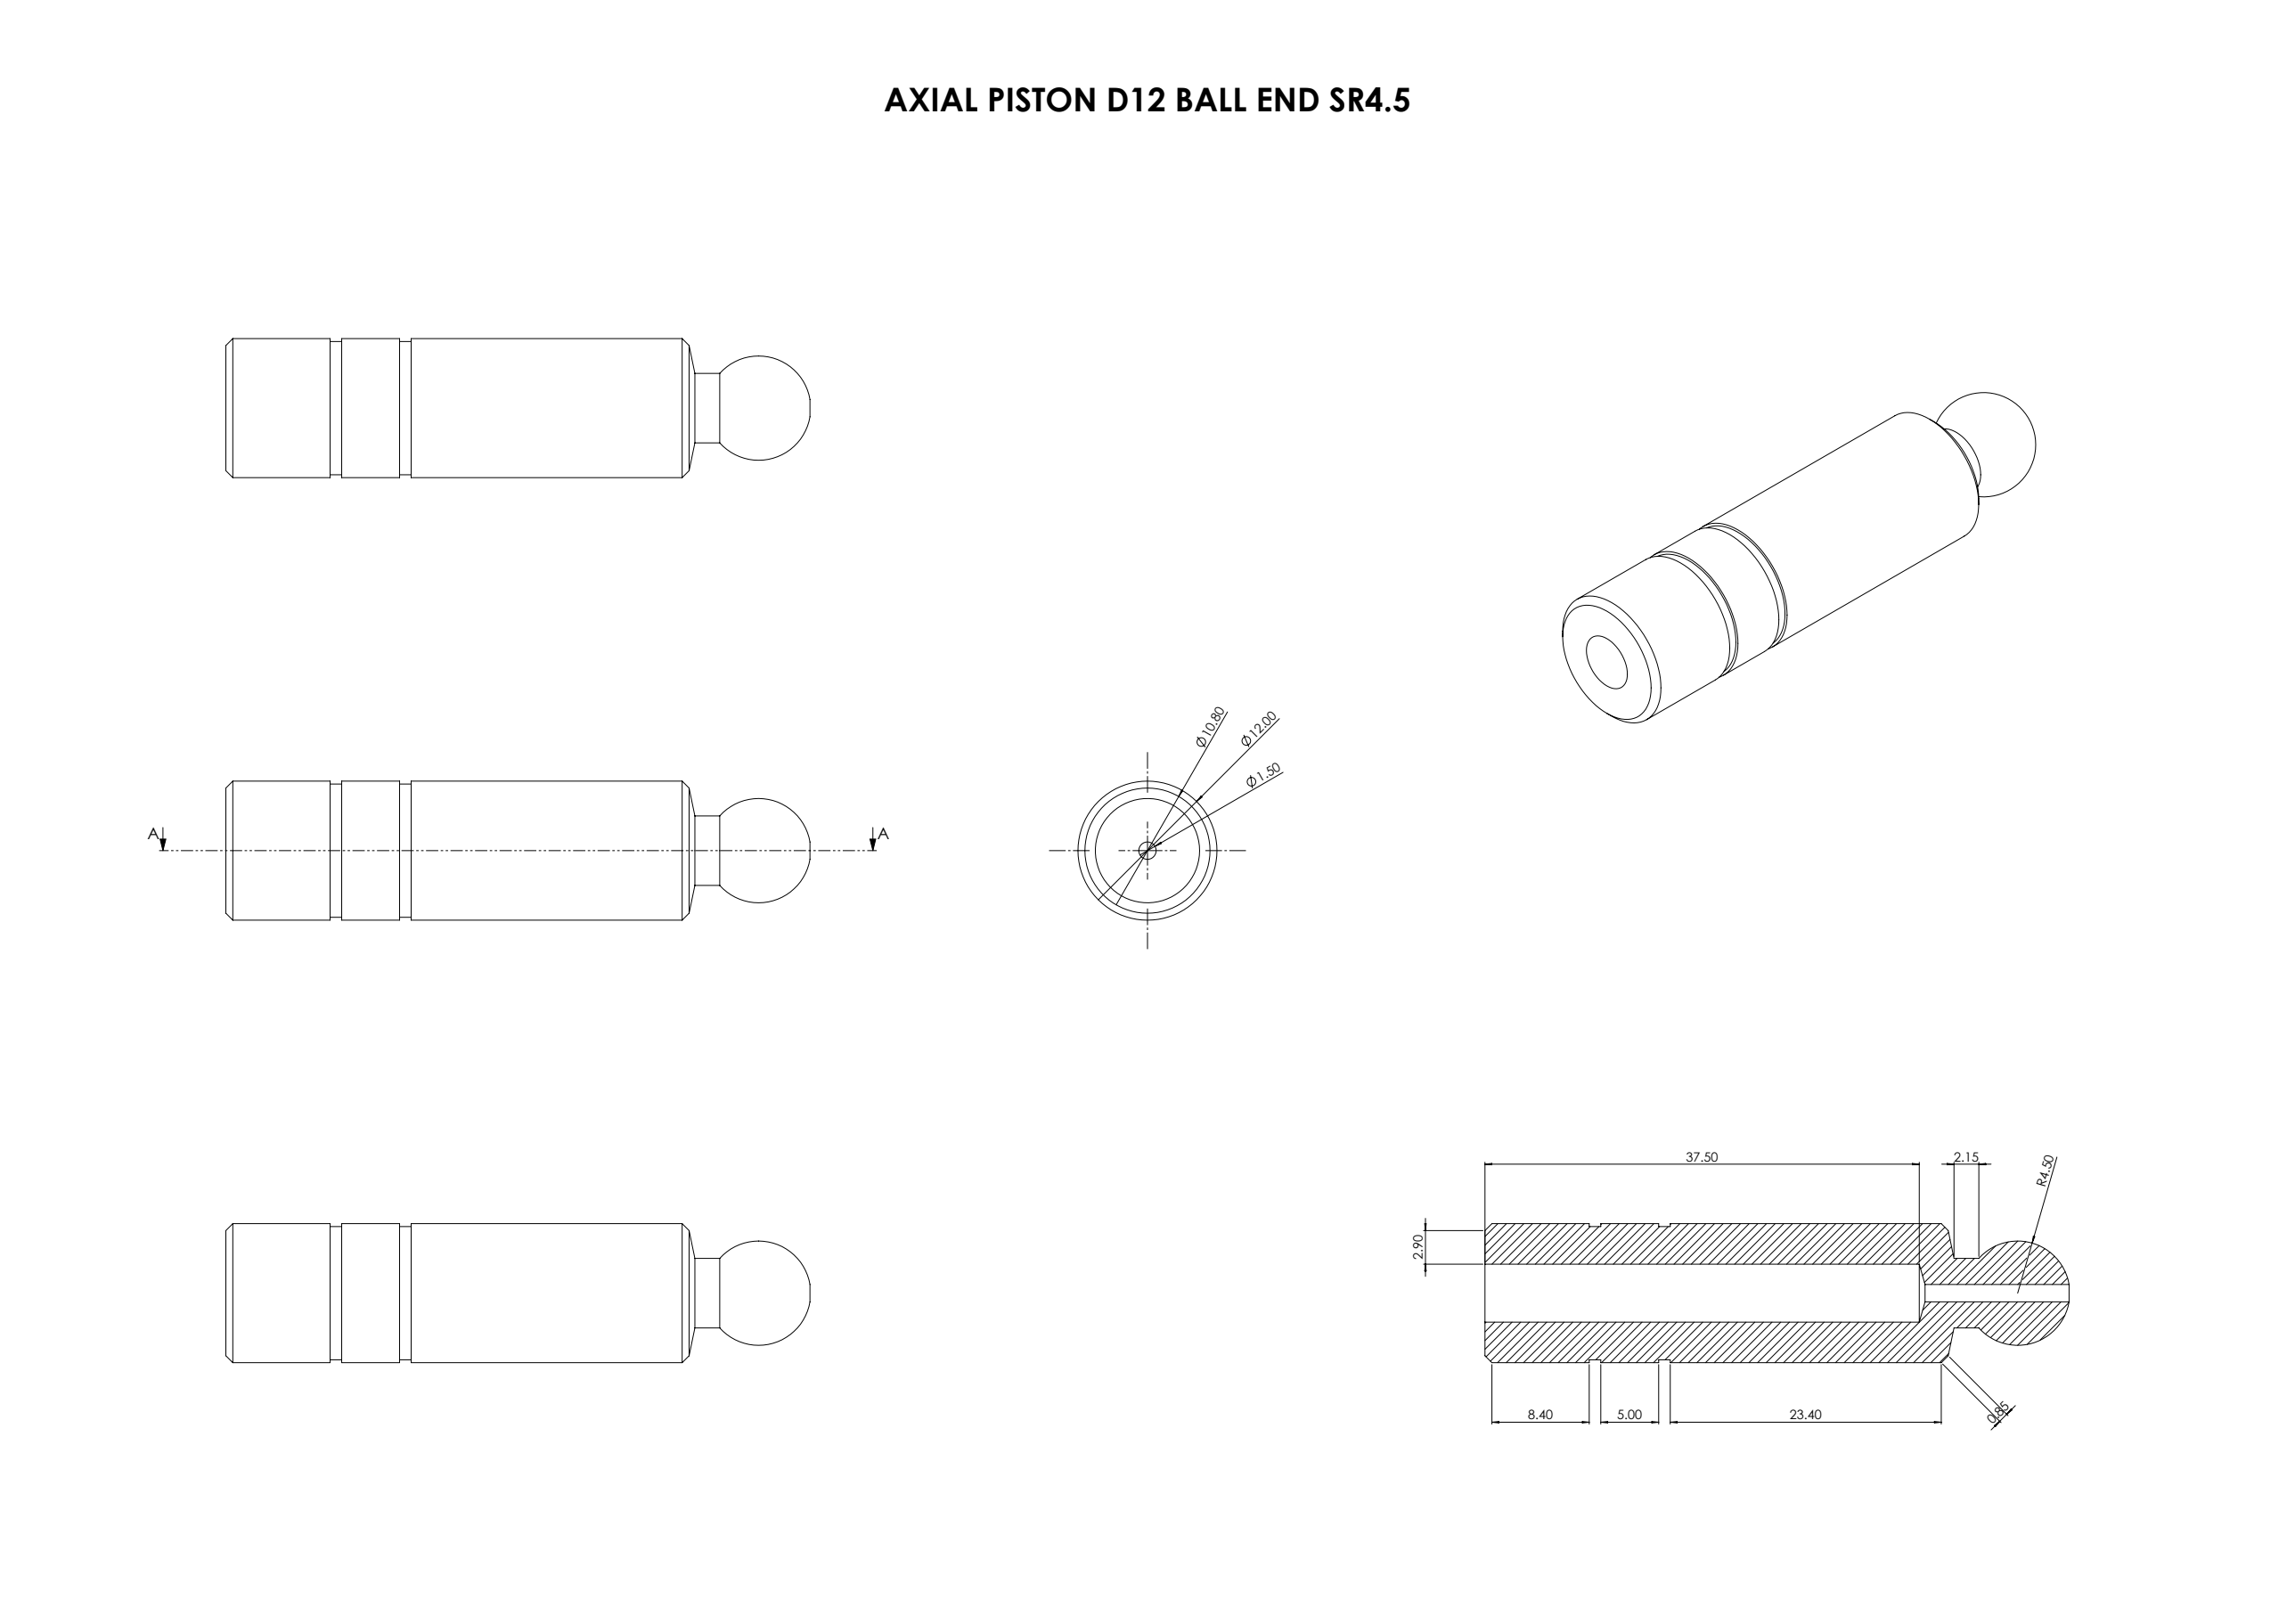
ISO-10303-21;
HEADER;
/* Generated by software containing ST-Developer
 * from STEP Tools, Inc. (www.steptools.com) 
 */

FILE_DESCRIPTION(
/* description */ (''),
/* implementation_level */ '2;1');

FILE_NAME(
/* name */ '06_Axial_Piston_D12_Ball_End_SR4.5.step',
/* time_stamp */ '2026-10-23T00:52:27+05:00',
/* author */ (''),
/* organization */ (''),
/* preprocessor_version */ 'ST-DEVELOPER v20.2',
/* originating_system */ 'Autodesk Translation Framework v15.15.0.0',
/* authorisation */ '');

FILE_SCHEMA (('AUTOMOTIVE_DESIGN { 1 0 10303 214 3 1 1 }'));
ENDSEC;

DATA;
#10=MECHANICAL_DESIGN_GEOMETRIC_PRESENTATION_REPRESENTATION('',(#1568),#59204);
#1521=SHAPE_REPRESENTATION_RELATIONSHIP('SRR','None',#59310,#1541);
#1541=ADVANCED_BREP_SHAPE_REPRESENTATION('',(#1588),#59197);
#1568=STYLED_ITEM('',(#59579),#1588);
#1588=MANIFOLD_SOLID_BREP('Piston',#22817);
#1597=SPHERICAL_SURFACE('',#24195,0.45);
#1747=FACE_BOUND('',#4969,.T.);
#1748=FACE_BOUND('',#4972,.T.);
#1749=FACE_BOUND('',#4975,.T.);
#1750=FACE_BOUND('',#4978,.T.);
#1751=FACE_BOUND('',#4986,.T.);
#2147=PLANE('',#24160);
#2148=PLANE('',#24165);
#2149=PLANE('',#24169);
#2150=PLANE('',#24173);
#2151=PLANE('',#24187);
#2565=CYLINDRICAL_SURFACE('',#24163,0.575);
#2566=CYLINDRICAL_SURFACE('',#24167,0.6);
#2567=CYLINDRICAL_SURFACE('',#24171,0.575);
#2568=CYLINDRICAL_SURFACE('',#24175,0.6);
#2569=CYLINDRICAL_SURFACE('',#24177,0.3);
#2570=CYLINDRICAL_SURFACE('',#24183,0.6);
#2571=CYLINDRICAL_SURFACE('',#24189,0.25);
#2572=CYLINDRICAL_SURFACE('',#24193,0.075);
#3515=FACE_OUTER_BOUND('',#4968,.T.);
#3516=FACE_OUTER_BOUND('',#4970,.T.);
#3517=FACE_OUTER_BOUND('',#4971,.T.);
#3518=FACE_OUTER_BOUND('',#4973,.T.);
#3519=FACE_OUTER_BOUND('',#4974,.T.);
#3520=FACE_OUTER_BOUND('',#4976,.T.);
#3521=FACE_OUTER_BOUND('',#4977,.T.);
#3522=FACE_OUTER_BOUND('',#4979,.T.);
#3523=FACE_OUTER_BOUND('',#4980,.T.);
#3524=FACE_OUTER_BOUND('',#4981,.T.);
#3525=FACE_OUTER_BOUND('',#4982,.T.);
#3526=FACE_OUTER_BOUND('',#4983,.T.);
#3527=FACE_OUTER_BOUND('',#4984,.T.);
#3528=FACE_OUTER_BOUND('',#4985,.T.);
#3529=FACE_OUTER_BOUND('',#4987,.T.);
#3530=FACE_OUTER_BOUND('',#4988,.T.);
#3531=FACE_OUTER_BOUND('',#4989,.T.);
#3532=FACE_OUTER_BOUND('',#4990,.T.);
#4968=EDGE_LOOP('',(#18954));
#4969=EDGE_LOOP('',(#18955));
#4970=EDGE_LOOP('',(#18956,#18957,#18958,#18959));
#4971=EDGE_LOOP('',(#18960));
#4972=EDGE_LOOP('',(#18961));
#4973=EDGE_LOOP('',(#18962,#18963,#18964,#18965));
#4974=EDGE_LOOP('',(#18966));
#4975=EDGE_LOOP('',(#18967));
#4976=EDGE_LOOP('',(#18968,#18969,#18970,#18971));
#4977=EDGE_LOOP('',(#18972));
#4978=EDGE_LOOP('',(#18973));
#4979=EDGE_LOOP('',(#18974,#18975,#18976,#18977));
#4980=EDGE_LOOP('',(#18978,#18979,#18980,#18981));
#4981=EDGE_LOOP('',(#18982,#18983,#18984,#18985));
#4982=EDGE_LOOP('',(#18986,#18987,#18988,#18989));
#4983=EDGE_LOOP('',(#18990,#18991,#18992,#18993));
#4984=EDGE_LOOP('',(#18994,#18995,#18996,#18997));
#4985=EDGE_LOOP('',(#18998));
#4986=EDGE_LOOP('',(#18999));
#4987=EDGE_LOOP('',(#19000,#19001,#19002,#19003));
#4988=EDGE_LOOP('',(#19004,#19005,#19006,#19007));
#4989=EDGE_LOOP('',(#19008,#19009,#19010,#19011));
#4990=EDGE_LOOP('',(#19012,#19013,#19014,#19015));
#6489=LINE('',#47284,#7922);
#6490=LINE('',#47290,#7923);
#6491=LINE('',#47298,#7924);
#6492=LINE('',#47304,#7925);
#6493=LINE('',#47310,#7926);
#6494=LINE('',#47315,#7927);
#6495=LINE('',#47317,#7928);
#6496=LINE('',#47321,#7929);
#6497=LINE('',#47325,#7930);
#6498=LINE('',#47331,#7931);
#6499=LINE('',#47335,#7932);
#6500=LINE('',#47339,#7933);
#7922=VECTOR('',#28355,0.575);
#7923=VECTOR('',#28362,0.6);
#7924=VECTOR('',#28373,0.575);
#7925=VECTOR('',#28380,0.6);
#7926=VECTOR('',#28387,0.3);
#7927=VECTOR('',#28394,0.42);
#7928=VECTOR('',#28397,0.57);
#7929=VECTOR('',#28402,0.6);
#7930=VECTOR('',#28407,0.57);
#7931=VECTOR('',#28414,0.25);
#7932=VECTOR('',#28419,0.1625);
#7933=VECTOR('',#28424,0.075);
#8855=CIRCLE('',#24161,0.6);
#8856=CIRCLE('',#24162,0.575);
#8857=CIRCLE('',#24164,0.575);
#8858=CIRCLE('',#24166,0.6);
#8859=CIRCLE('',#24168,0.6);
#8860=CIRCLE('',#24170,0.575);
#8861=CIRCLE('',#24172,0.575);
#8862=CIRCLE('',#24174,0.6);
#8863=CIRCLE('',#24176,0.6);
#8864=CIRCLE('',#24178,0.3);
#8865=CIRCLE('',#24179,0.3);
#8866=CIRCLE('',#24181,0.54);
#8867=CIRCLE('',#24184,0.6);
#8868=CIRCLE('',#24186,0.54);
#8869=CIRCLE('',#24188,0.25);
#8870=CIRCLE('',#24190,0.25);
#8871=CIRCLE('',#24192,0.075);
#8872=CIRCLE('',#24194,0.075);
#8873=CIRCLE('',#24196,0.45);
#10582=VERTEX_POINT('',#47277);
#10583=VERTEX_POINT('',#47279);
#10584=VERTEX_POINT('',#47282);
#10585=VERTEX_POINT('',#47286);
#10586=VERTEX_POINT('',#47289);
#10587=VERTEX_POINT('',#47293);
#10588=VERTEX_POINT('',#47296);
#10589=VERTEX_POINT('',#47300);
#10590=VERTEX_POINT('',#47303);
#10591=VERTEX_POINT('',#47307);
#10592=VERTEX_POINT('',#47309);
#10593=VERTEX_POINT('',#47313);
#10594=VERTEX_POINT('',#47319);
#10595=VERTEX_POINT('',#47323);
#10596=VERTEX_POINT('',#47327);
#10597=VERTEX_POINT('',#47330);
#10598=VERTEX_POINT('',#47334);
#10599=VERTEX_POINT('',#47338);
#13481=EDGE_CURVE('',#10582,#10582,#8855,.T.);
#13482=EDGE_CURVE('',#10583,#10583,#8856,.T.);
#13483=EDGE_CURVE('',#10584,#10584,#8857,.T.);
#13484=EDGE_CURVE('',#10584,#10583,#6489,.T.);
#13485=EDGE_CURVE('',#10585,#10585,#8858,.T.);
#13486=EDGE_CURVE('',#10585,#10586,#6490,.T.);
#13487=EDGE_CURVE('',#10586,#10586,#8859,.T.);
#13488=EDGE_CURVE('',#10587,#10587,#8860,.T.);
#13489=EDGE_CURVE('',#10588,#10588,#8861,.T.);
#13490=EDGE_CURVE('',#10588,#10587,#6491,.T.);
#13491=EDGE_CURVE('',#10589,#10589,#8862,.T.);
#13492=EDGE_CURVE('',#10589,#10590,#6492,.T.);
#13493=EDGE_CURVE('',#10590,#10590,#8863,.T.);
#13494=EDGE_CURVE('',#10591,#10591,#8864,.T.);
#13495=EDGE_CURVE('',#10591,#10592,#6493,.T.);
#13496=EDGE_CURVE('',#10592,#10592,#8865,.T.);
#13497=EDGE_CURVE('',#10593,#10593,#8866,.T.);
#13498=EDGE_CURVE('',#10593,#10591,#6494,.T.);
#13499=EDGE_CURVE('',#10590,#10593,#6495,.T.);
#13500=EDGE_CURVE('',#10594,#10594,#8867,.T.);
#13501=EDGE_CURVE('',#10594,#10582,#6496,.T.);
#13502=EDGE_CURVE('',#10595,#10595,#8868,.T.);
#13503=EDGE_CURVE('',#10595,#10594,#6497,.T.);
#13504=EDGE_CURVE('',#10596,#10596,#8869,.T.);
#13505=EDGE_CURVE('',#10596,#10597,#6498,.T.);
#13506=EDGE_CURVE('',#10597,#10597,#8870,.T.);
#13507=EDGE_CURVE('',#10597,#10598,#6499,.T.);
#13508=EDGE_CURVE('',#10598,#10598,#8871,.T.);
#13509=EDGE_CURVE('',#10598,#10599,#6500,.T.);
#13510=EDGE_CURVE('',#10599,#10599,#8872,.T.);
#13511=EDGE_CURVE('',#10592,#10599,#8873,.T.);
#18954=ORIENTED_EDGE('',*,*,#13481,.F.);
#18955=ORIENTED_EDGE('',*,*,#13482,.T.);
#18956=ORIENTED_EDGE('',*,*,#13483,.T.);
#18957=ORIENTED_EDGE('',*,*,#13484,.T.);
#18958=ORIENTED_EDGE('',*,*,#13482,.F.);
#18959=ORIENTED_EDGE('',*,*,#13484,.F.);
#18960=ORIENTED_EDGE('',*,*,#13485,.F.);
#18961=ORIENTED_EDGE('',*,*,#13483,.F.);
#18962=ORIENTED_EDGE('',*,*,#13485,.T.);
#18963=ORIENTED_EDGE('',*,*,#13486,.T.);
#18964=ORIENTED_EDGE('',*,*,#13487,.T.);
#18965=ORIENTED_EDGE('',*,*,#13486,.F.);
#18966=ORIENTED_EDGE('',*,*,#13487,.F.);
#18967=ORIENTED_EDGE('',*,*,#13488,.T.);
#18968=ORIENTED_EDGE('',*,*,#13489,.T.);
#18969=ORIENTED_EDGE('',*,*,#13490,.T.);
#18970=ORIENTED_EDGE('',*,*,#13488,.F.);
#18971=ORIENTED_EDGE('',*,*,#13490,.F.);
#18972=ORIENTED_EDGE('',*,*,#13491,.F.);
#18973=ORIENTED_EDGE('',*,*,#13489,.F.);
#18974=ORIENTED_EDGE('',*,*,#13491,.T.);
#18975=ORIENTED_EDGE('',*,*,#13492,.T.);
#18976=ORIENTED_EDGE('',*,*,#13493,.T.);
#18977=ORIENTED_EDGE('',*,*,#13492,.F.);
#18978=ORIENTED_EDGE('',*,*,#13494,.F.);
#18979=ORIENTED_EDGE('',*,*,#13495,.T.);
#18980=ORIENTED_EDGE('',*,*,#13496,.T.);
#18981=ORIENTED_EDGE('',*,*,#13495,.F.);
#18982=ORIENTED_EDGE('',*,*,#13497,.F.);
#18983=ORIENTED_EDGE('',*,*,#13498,.T.);
#18984=ORIENTED_EDGE('',*,*,#13494,.T.);
#18985=ORIENTED_EDGE('',*,*,#13498,.F.);
#18986=ORIENTED_EDGE('',*,*,#13493,.F.);
#18987=ORIENTED_EDGE('',*,*,#13499,.T.);
#18988=ORIENTED_EDGE('',*,*,#13497,.T.);
#18989=ORIENTED_EDGE('',*,*,#13499,.F.);
#18990=ORIENTED_EDGE('',*,*,#13500,.F.);
#18991=ORIENTED_EDGE('',*,*,#13501,.T.);
#18992=ORIENTED_EDGE('',*,*,#13481,.T.);
#18993=ORIENTED_EDGE('',*,*,#13501,.F.);
#18994=ORIENTED_EDGE('',*,*,#13502,.F.);
#18995=ORIENTED_EDGE('',*,*,#13503,.T.);
#18996=ORIENTED_EDGE('',*,*,#13500,.T.);
#18997=ORIENTED_EDGE('',*,*,#13503,.F.);
#18998=ORIENTED_EDGE('',*,*,#13502,.T.);
#18999=ORIENTED_EDGE('',*,*,#13504,.F.);
#19000=ORIENTED_EDGE('',*,*,#13504,.T.);
#19001=ORIENTED_EDGE('',*,*,#13505,.T.);
#19002=ORIENTED_EDGE('',*,*,#13506,.F.);
#19003=ORIENTED_EDGE('',*,*,#13505,.F.);
#19004=ORIENTED_EDGE('',*,*,#13506,.T.);
#19005=ORIENTED_EDGE('',*,*,#13507,.T.);
#19006=ORIENTED_EDGE('',*,*,#13508,.F.);
#19007=ORIENTED_EDGE('',*,*,#13507,.F.);
#19008=ORIENTED_EDGE('',*,*,#13508,.T.);
#19009=ORIENTED_EDGE('',*,*,#13509,.T.);
#19010=ORIENTED_EDGE('',*,*,#13510,.F.);
#19011=ORIENTED_EDGE('',*,*,#13509,.F.);
#19012=ORIENTED_EDGE('',*,*,#13496,.F.);
#19013=ORIENTED_EDGE('',*,*,#13511,.T.);
#19014=ORIENTED_EDGE('',*,*,#13510,.T.);
#19015=ORIENTED_EDGE('',*,*,#13511,.F.);
#21419=CONICAL_SURFACE('',#24180,0.42,1.36540093760513);
#21420=CONICAL_SURFACE('',#24182,0.57,0.785398163397448);
#21421=CONICAL_SURFACE('',#24185,0.57,0.785398163397451);
#21422=CONICAL_SURFACE('',#24191,0.1625,1.29249666778979);
#22345=ADVANCED_FACE('',(#3515,#1747),#2147,.F.);
#22346=ADVANCED_FACE('',(#3516),#2565,.T.);
#22347=ADVANCED_FACE('',(#3517,#1748),#2148,.F.);
#22348=ADVANCED_FACE('',(#3518),#2566,.T.);
#22349=ADVANCED_FACE('',(#3519,#1749),#2149,.F.);
#22350=ADVANCED_FACE('',(#3520),#2567,.T.);
#22351=ADVANCED_FACE('',(#3521,#1750),#2150,.F.);
#22352=ADVANCED_FACE('',(#3522),#2568,.T.);
#22353=ADVANCED_FACE('',(#3523),#2569,.T.);
#22354=ADVANCED_FACE('',(#3524),#21419,.T.);
#22355=ADVANCED_FACE('',(#3525),#21420,.T.);
#22356=ADVANCED_FACE('',(#3526),#2570,.T.);
#22357=ADVANCED_FACE('',(#3527),#21421,.T.);
#22358=ADVANCED_FACE('',(#3528,#1751),#2151,.T.);
#22359=ADVANCED_FACE('',(#3529),#2571,.F.);
#22360=ADVANCED_FACE('',(#3530),#21422,.F.);
#22361=ADVANCED_FACE('',(#3531),#2572,.F.);
#22362=ADVANCED_FACE('',(#3532),#1597,.T.);
#22817=CLOSED_SHELL('',(#22345,#22346,#22347,#22348,#22349,#22350,#22351,
#22352,#22353,#22354,#22355,#22356,#22357,#22358,#22359,#22360,#22361,#22362));
#24159=AXIS2_PLACEMENT_3D('',#47275,#28343,#28344);
#24160=AXIS2_PLACEMENT_3D('',#47276,#28345,#28346);
#24161=AXIS2_PLACEMENT_3D('',#47278,#28347,#28348);
#24162=AXIS2_PLACEMENT_3D('',#47280,#28349,#28350);
#24163=AXIS2_PLACEMENT_3D('',#47281,#28351,#28352);
#24164=AXIS2_PLACEMENT_3D('',#47283,#28353,#28354);
#24165=AXIS2_PLACEMENT_3D('',#47285,#28356,#28357);
#24166=AXIS2_PLACEMENT_3D('',#47287,#28358,#28359);
#24167=AXIS2_PLACEMENT_3D('',#47288,#28360,#28361);
#24168=AXIS2_PLACEMENT_3D('',#47291,#28363,#28364);
#24169=AXIS2_PLACEMENT_3D('',#47292,#28365,#28366);
#24170=AXIS2_PLACEMENT_3D('',#47294,#28367,#28368);
#24171=AXIS2_PLACEMENT_3D('',#47295,#28369,#28370);
#24172=AXIS2_PLACEMENT_3D('',#47297,#28371,#28372);
#24173=AXIS2_PLACEMENT_3D('',#47299,#28374,#28375);
#24174=AXIS2_PLACEMENT_3D('',#47301,#28376,#28377);
#24175=AXIS2_PLACEMENT_3D('',#47302,#28378,#28379);
#24176=AXIS2_PLACEMENT_3D('',#47305,#28381,#28382);
#24177=AXIS2_PLACEMENT_3D('',#47306,#28383,#28384);
#24178=AXIS2_PLACEMENT_3D('',#47308,#28385,#28386);
#24179=AXIS2_PLACEMENT_3D('',#47311,#28388,#28389);
#24180=AXIS2_PLACEMENT_3D('',#47312,#28390,#28391);
#24181=AXIS2_PLACEMENT_3D('',#47314,#28392,#28393);
#24182=AXIS2_PLACEMENT_3D('',#47316,#28395,#28396);
#24183=AXIS2_PLACEMENT_3D('',#47318,#28398,#28399);
#24184=AXIS2_PLACEMENT_3D('',#47320,#28400,#28401);
#24185=AXIS2_PLACEMENT_3D('',#47322,#28403,#28404);
#24186=AXIS2_PLACEMENT_3D('',#47324,#28405,#28406);
#24187=AXIS2_PLACEMENT_3D('',#47326,#28408,#28409);
#24188=AXIS2_PLACEMENT_3D('',#47328,#28410,#28411);
#24189=AXIS2_PLACEMENT_3D('',#47329,#28412,#28413);
#24190=AXIS2_PLACEMENT_3D('',#47332,#28415,#28416);
#24191=AXIS2_PLACEMENT_3D('',#47333,#28417,#28418);
#24192=AXIS2_PLACEMENT_3D('',#47336,#28420,#28421);
#24193=AXIS2_PLACEMENT_3D('',#47337,#28422,#28423);
#24194=AXIS2_PLACEMENT_3D('',#47340,#28425,#28426);
#24195=AXIS2_PLACEMENT_3D('',#47341,#28427,#28428);
#24196=AXIS2_PLACEMENT_3D('',#47342,#28429,#28430);
#28343=DIRECTION('axis',(0.,0.,1.));
#28344=DIRECTION('refdir',(1.,0.,0.));
#28345=DIRECTION('center_axis',(0.,0.,1.));
#28346=DIRECTION('ref_axis',(1.,0.,0.));
#28347=DIRECTION('center_axis',(0.,0.,1.));
#28348=DIRECTION('ref_axis',(1.,0.,0.));
#28349=DIRECTION('center_axis',(0.,0.,1.));
#28350=DIRECTION('ref_axis',(1.,0.,0.));
#28351=DIRECTION('center_axis',(0.,0.,1.));
#28352=DIRECTION('ref_axis',(1.,0.,0.));
#28353=DIRECTION('center_axis',(0.,0.,1.));
#28354=DIRECTION('ref_axis',(1.,0.,0.));
#28355=DIRECTION('',(0.,0.,1.));
#28356=DIRECTION('center_axis',(0.,0.,-1.));
#28357=DIRECTION('ref_axis',(-1.,0.,0.));
#28358=DIRECTION('center_axis',(0.,0.,-1.));
#28359=DIRECTION('ref_axis',(1.,0.,0.));
#28360=DIRECTION('center_axis',(0.,0.,1.));
#28361=DIRECTION('ref_axis',(1.,0.,0.));
#28362=DIRECTION('',(0.,0.,-1.));
#28363=DIRECTION('center_axis',(0.,0.,1.));
#28364=DIRECTION('ref_axis',(1.,0.,0.));
#28365=DIRECTION('center_axis',(0.,0.,1.));
#28366=DIRECTION('ref_axis',(1.,0.,0.));
#28367=DIRECTION('center_axis',(0.,0.,1.));
#28368=DIRECTION('ref_axis',(1.,0.,0.));
#28369=DIRECTION('center_axis',(0.,0.,1.));
#28370=DIRECTION('ref_axis',(1.,0.,0.));
#28371=DIRECTION('center_axis',(0.,0.,1.));
#28372=DIRECTION('ref_axis',(1.,0.,0.));
#28373=DIRECTION('',(0.,0.,1.));
#28374=DIRECTION('center_axis',(0.,0.,-1.));
#28375=DIRECTION('ref_axis',(-1.,0.,0.));
#28376=DIRECTION('center_axis',(0.,0.,-1.));
#28377=DIRECTION('ref_axis',(1.,0.,0.));
#28378=DIRECTION('center_axis',(0.,0.,1.));
#28379=DIRECTION('ref_axis',(1.,0.,0.));
#28380=DIRECTION('',(0.,0.,-1.));
#28381=DIRECTION('center_axis',(0.,0.,1.));
#28382=DIRECTION('ref_axis',(1.,0.,0.));
#28383=DIRECTION('center_axis',(0.,0.,1.));
#28384=DIRECTION('ref_axis',(1.,0.,0.));
#28385=DIRECTION('center_axis',(0.,0.,1.));
#28386=DIRECTION('ref_axis',(1.,0.,0.));
#28387=DIRECTION('',(0.,0.,-1.));
#28388=DIRECTION('center_axis',(0.,0.,1.));
#28389=DIRECTION('ref_axis',(1.,0.,0.));
#28390=DIRECTION('center_axis',(0.,0.,1.));
#28391=DIRECTION('ref_axis',(1.,0.,0.));
#28392=DIRECTION('center_axis',(0.,0.,1.));
#28393=DIRECTION('ref_axis',(1.,0.,0.));
#28394=DIRECTION('',(0.978980419737605,1.19890523745959E-16,-0.203954254112001));
#28395=DIRECTION('center_axis',(0.,0.,1.));
#28396=DIRECTION('ref_axis',(1.,0.,0.));
#28397=DIRECTION('',(0.707106781186548,8.65956056235493E-17,-0.707106781186547));
#28398=DIRECTION('center_axis',(0.,0.,1.));
#28399=DIRECTION('ref_axis',(1.,0.,0.));
#28400=DIRECTION('center_axis',(0.,0.,1.));
#28401=DIRECTION('ref_axis',(1.,0.,0.));
#28402=DIRECTION('',(0.,0.,-1.));
#28403=DIRECTION('center_axis',(0.,0.,-1.));
#28404=DIRECTION('ref_axis',(1.,0.,0.));
#28405=DIRECTION('center_axis',(0.,0.,1.));
#28406=DIRECTION('ref_axis',(1.,0.,0.));
#28407=DIRECTION('',(-0.707106781186549,-8.65956056235496E-17,-0.707106781186546));
#28408=DIRECTION('center_axis',(0.,0.,1.));
#28409=DIRECTION('ref_axis',(1.,0.,0.));
#28410=DIRECTION('center_axis',(0.,0.,1.));
#28411=DIRECTION('ref_axis',(1.,0.,0.));
#28412=DIRECTION('center_axis',(0.,0.,1.));
#28413=DIRECTION('ref_axis',(1.,0.,0.));
#28414=DIRECTION('',(0.,0.,-1.));
#28415=DIRECTION('center_axis',(0.,0.,1.));
#28416=DIRECTION('ref_axis',(1.,0.,0.));
#28417=DIRECTION('center_axis',(0.,0.,1.));
#28418=DIRECTION('ref_axis',(1.,0.,0.));
#28419=DIRECTION('',(0.961523947640823,1.17752722478186E-16,-0.274721127897378));
#28420=DIRECTION('center_axis',(0.,0.,1.));
#28421=DIRECTION('ref_axis',(1.,0.,0.));
#28422=DIRECTION('center_axis',(0.,0.,1.));
#28423=DIRECTION('ref_axis',(1.,0.,0.));
#28424=DIRECTION('',(0.,0.,-1.));
#28425=DIRECTION('center_axis',(0.,0.,1.));
#28426=DIRECTION('ref_axis',(1.,0.,0.));
#28427=DIRECTION('center_axis',(6.12323399573677E-17,0.,1.));
#28428=DIRECTION('ref_axis',(1.,0.,0.));
#28429=DIRECTION('center_axis',(1.22464679914735E-16,-1.,0.));
#28430=DIRECTION('ref_axis',(-1.,-1.22464679914735E-16,0.));
#47275=CARTESIAN_POINT('',(0.,0.,0.));
#47276=CARTESIAN_POINT('Origin',(0.575,0.,3.7));
#47277=CARTESIAN_POINT('',(-0.6,-7.34788079488412E-17,3.7));
#47278=CARTESIAN_POINT('Origin',(0.,0.,3.7));
#47279=CARTESIAN_POINT('',(-0.575,-7.04171909509728E-17,3.7));
#47280=CARTESIAN_POINT('Origin',(0.,0.,3.7));
#47281=CARTESIAN_POINT('Origin',(0.,0.,3.65));
#47282=CARTESIAN_POINT('',(-0.575,-7.04171909509728E-17,3.6));
#47283=CARTESIAN_POINT('Origin',(0.,0.,3.6));
#47284=CARTESIAN_POINT('',(-0.575,-7.04171909509728E-17,3.65));
#47285=CARTESIAN_POINT('Origin',(0.61,0.,3.6));
#47286=CARTESIAN_POINT('',(-0.6,7.34788079488412E-17,3.6));
#47287=CARTESIAN_POINT('Origin',(0.,0.,3.6));
#47288=CARTESIAN_POINT('Origin',(0.,0.,2.6));
#47289=CARTESIAN_POINT('',(-0.6,-7.34788079488412E-17,3.1));
#47290=CARTESIAN_POINT('',(-0.6,-7.34788079488412E-17,2.6));
#47291=CARTESIAN_POINT('Origin',(0.,0.,3.1));
#47292=CARTESIAN_POINT('Origin',(0.575,0.,3.1));
#47293=CARTESIAN_POINT('',(-0.575,-7.04171909509728E-17,3.1));
#47294=CARTESIAN_POINT('Origin',(0.,0.,3.1));
#47295=CARTESIAN_POINT('Origin',(0.,0.,3.05));
#47296=CARTESIAN_POINT('',(-0.575,-7.04171909509728E-17,3.));
#47297=CARTESIAN_POINT('Origin',(0.,0.,3.));
#47298=CARTESIAN_POINT('',(-0.575,-7.04171909509728E-17,3.05));
#47299=CARTESIAN_POINT('Origin',(0.61,0.,3.));
#47300=CARTESIAN_POINT('',(-0.6,7.34788079488412E-17,3.));
#47301=CARTESIAN_POINT('Origin',(0.,0.,3.));
#47302=CARTESIAN_POINT('Origin',(0.,0.,2.6));
#47303=CARTESIAN_POINT('',(-0.6,-7.34788079488412E-17,0.66));
#47304=CARTESIAN_POINT('',(-0.6,-7.34788079488412E-17,2.6));
#47305=CARTESIAN_POINT('Origin',(0.,0.,0.66));
#47306=CARTESIAN_POINT('Origin',(0.,0.,0.442705098312484));
#47307=CARTESIAN_POINT('',(-0.3,-3.67394039744206E-17,0.55));
#47308=CARTESIAN_POINT('Origin',(0.,0.,0.55));
#47309=CARTESIAN_POINT('',(-0.3,-3.67394039744206E-17,0.335410196624968));
#47310=CARTESIAN_POINT('',(-0.3,-3.67394039744206E-17,0.442705098312484));
#47311=CARTESIAN_POINT('Origin',(0.,0.,0.335410196624968));
#47312=CARTESIAN_POINT('Origin',(0.,0.,0.575));
#47313=CARTESIAN_POINT('',(-0.54,-6.61309271539571E-17,0.6));
#47314=CARTESIAN_POINT('Origin',(0.,0.,0.6));
#47315=CARTESIAN_POINT('',(-0.42,-5.14351655641888E-17,0.575));
#47316=CARTESIAN_POINT('Origin',(0.,0.,0.63));
#47317=CARTESIAN_POINT('',(-0.57,-6.98048675513991E-17,0.63));
#47318=CARTESIAN_POINT('Origin',(0.,0.,2.6));
#47319=CARTESIAN_POINT('',(-0.6,-7.34788079488412E-17,4.54));
#47320=CARTESIAN_POINT('Origin',(0.,0.,4.54));
#47321=CARTESIAN_POINT('',(-0.6,-7.34788079488412E-17,2.6));
#47322=CARTESIAN_POINT('Origin',(0.,0.,4.57));
#47323=CARTESIAN_POINT('',(-0.54,-6.61309271539571E-17,4.6));
#47324=CARTESIAN_POINT('Origin',(0.,0.,4.6));
#47325=CARTESIAN_POINT('',(-0.57,-6.98048675513991E-17,4.57));
#47326=CARTESIAN_POINT('Origin',(0.25,0.,4.6));
#47327=CARTESIAN_POINT('',(-0.25,-3.06161699786838E-17,4.6));
#47328=CARTESIAN_POINT('Origin',(0.,0.,4.6));
#47329=CARTESIAN_POINT('Origin',(0.,0.,2.725));
#47330=CARTESIAN_POINT('',(-0.25,-3.06161699786838E-17,0.85));
#47331=CARTESIAN_POINT('',(-0.25,-3.06161699786838E-17,2.725));
#47332=CARTESIAN_POINT('Origin',(0.,0.,0.85));
#47333=CARTESIAN_POINT('Origin',(0.,0.,0.825));
#47334=CARTESIAN_POINT('',(-0.075,-9.18485099360515E-18,0.8));
#47335=CARTESIAN_POINT('',(-0.1625,-1.99005104861445E-17,0.825));
#47336=CARTESIAN_POINT('Origin',(0.,0.,0.8));
#47337=CARTESIAN_POINT('Origin',(0.,0.,0.178147008133764));
#47338=CARTESIAN_POINT('',(-0.075,-9.18485099360515E-18,-0.443705983732471));
#47339=CARTESIAN_POINT('',(-0.075,-9.18485099360515E-18,0.178147008133764));
#47340=CARTESIAN_POINT('Origin',(0.,0.,-0.443705983732471));
#47341=CARTESIAN_POINT('Origin',(0.,0.,0.));
#47342=CARTESIAN_POINT('Origin',(0.,0.,0.));
#59175=UNCERTAINTY_MEASURE_WITH_UNIT(LENGTH_MEASURE(0.001),#59205,
'DISTANCE_ACCURACY_VALUE',
'Maximum model space distance between geometric entities at asserted c
onnectivities');
#59182=UNCERTAINTY_MEASURE_WITH_UNIT(LENGTH_MEASURE(0.001),#59205,
'DISTANCE_ACCURACY_VALUE',
'Maximum model space distance between geometric entities at asserted c
onnectivities');
#59197=(
GEOMETRIC_REPRESENTATION_CONTEXT(3)
GLOBAL_UNCERTAINTY_ASSIGNED_CONTEXT((#59175))
GLOBAL_UNIT_ASSIGNED_CONTEXT((#59205,#59207,#59208))
REPRESENTATION_CONTEXT('','3D')
);
#59204=(
GEOMETRIC_REPRESENTATION_CONTEXT(3)
GLOBAL_UNCERTAINTY_ASSIGNED_CONTEXT((#59182))
GLOBAL_UNIT_ASSIGNED_CONTEXT((#59205,#59207,#59208))
REPRESENTATION_CONTEXT('','3D')
);
#59205=(
LENGTH_UNIT()
NAMED_UNIT(*)
SI_UNIT(.CENTI.,.METRE.)
);
#59207=(
NAMED_UNIT(*)
PLANE_ANGLE_UNIT()
SI_UNIT($,.RADIAN.)
);
#59208=(
NAMED_UNIT(*)
SI_UNIT($,.STERADIAN.)
SOLID_ANGLE_UNIT()
);
#59223=SHAPE_DEFINITION_REPRESENTATION(#59244,#59310);
#59244=PRODUCT_DEFINITION_SHAPE('',$,#59332);
#59310=SHAPE_REPRESENTATION('',(#24159),#59197);
#59317=PRODUCT_DEFINITION_CONTEXT('part definition',#59382,'design');
#59332=PRODUCT_DEFINITION('2026-10-23-00-47-08-320',
'06_Axial_Piston_D12_Ball_End_SR4.5',#59353,#59317);
#59353=PRODUCT_DEFINITION_FORMATION('',$,#59398);
#59382=APPLICATION_CONTEXT(
'Core Data for Automotive Mechanical Design Process');
#59383=PRODUCT_CONTEXT('part definition',#59382,'mechanical');
#59398=PRODUCT('2026-10-23-00-47-08-320',
'06_Axial_Piston_D12_Ball_End_SR4.5',$,(#59383));
#59573=COLOUR_RGB('Sky Blue',0.24,0.69,0.87);
#59574=FILL_AREA_STYLE_COLOUR('',#59573);
#59575=FILL_AREA_STYLE('',(#59574));
#59576=SURFACE_STYLE_FILL_AREA(#59575);
#59577=SURFACE_SIDE_STYLE('',(#59576));
#59578=SURFACE_STYLE_USAGE(.BOTH.,#59577);
#59579=PRESENTATION_STYLE_ASSIGNMENT((#59578));
ENDSEC;
END-ISO-10303-21;
